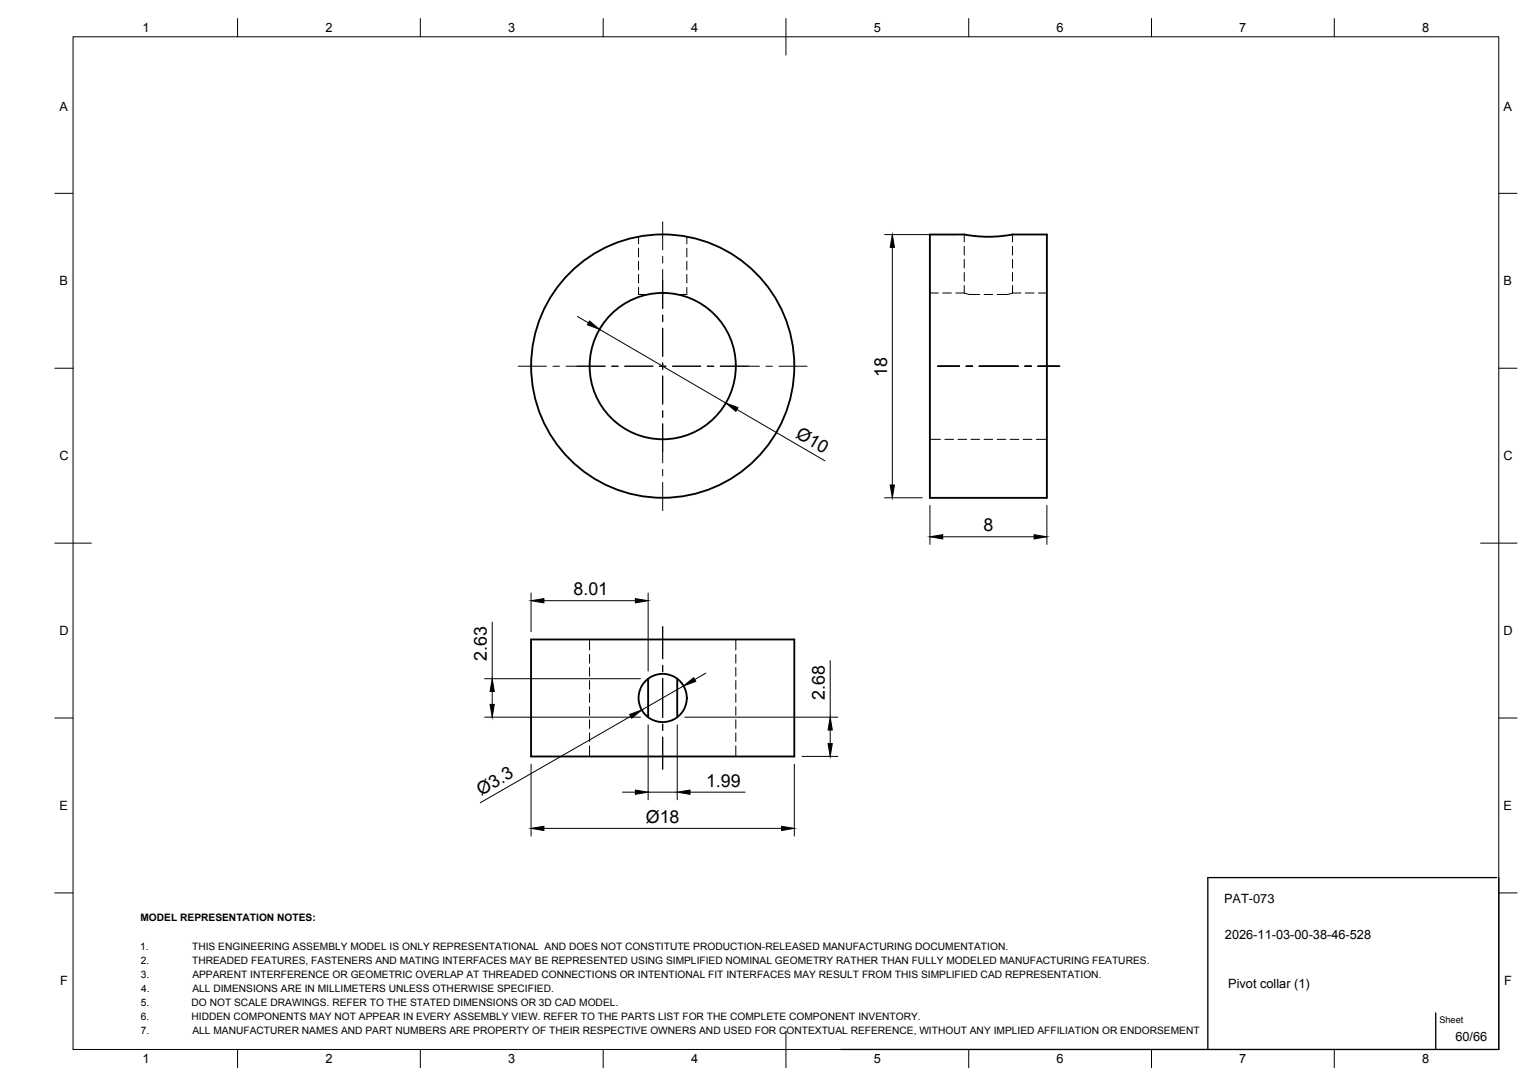
ISO-10303-21;
HEADER;
/* Generated by software containing ST-Developer
 * from STEP Tools, Inc. (www.steptools.com) 
 */

FILE_DESCRIPTION(
/* description */ ('Manual piston pump'),
/* implementation_level */ '2;1');

FILE_NAME(
/* name */ 'Pivot collar (1).step',
/* time_stamp */ '2026-11-02T16:54:23-08:00',
/* author */ (''),
/* organization */ (''),
/* preprocessor_version */ 'ST-DEVELOPER v20.2',
/* originating_system */ 'Autodesk Translation Framework v15.17.0.0',
/* authorisation */ '');

FILE_SCHEMA (('AUTOMOTIVE_DESIGN { 1 0 10303 214 3 1 1 }'));
ENDSEC;

DATA;
#10=MECHANICAL_DESIGN_GEOMETRIC_PRESENTATION_REPRESENTATION('',(#750),#19043);
#616=SHAPE_REPRESENTATION_RELATIONSHIP('SRR','None',#19366,#679);
#679=ADVANCED_BREP_SHAPE_REPRESENTATION('',(#818),#19033);
#750=STYLED_ITEM('',(#19661),#818);
#818=MANIFOLD_SOLID_BREP('Body1',#9538);
#1030=FACE_BOUND('',#2573,.T.);
#1031=FACE_BOUND('',#2575,.T.);
#1084=B_SPLINE_CURVE_WITH_KNOTS('',3,(#18479,#18480,#18481,#18482,#18483,
#18484),.UNSPECIFIED.,.F.,.F.,(4,2,4),(0.649292020015395,0.689320963667327,
0.7519713082482),.UNSPECIFIED.);
#1085=B_SPLINE_CURVE_WITH_KNOTS('',3,(#18488,#18489,#18490,#18491,#18492,
#18493),.UNSPECIFIED.,.F.,.F.,(4,2,4),(0.2506571027494,0.313307447330273,
0.353336390982205),.UNSPECIFIED.);
#1086=B_SPLINE_CURVE_WITH_KNOTS('',3,(#18494,#18495,#18496,#18497,#18498,
#18499),.UNSPECIFIED.,.F.,.F.,(4,2,4),(0.147977814516595,0.188006758168527,
0.2506571027494),.UNSPECIFIED.);
#1087=B_SPLINE_CURVE_WITH_KNOTS('',3,(#18500,#18501,#18502,#18503,#18504,
#18505),.UNSPECIFIED.,.F.,.F.,(4,2,4),(0.7519713082482,0.814621652829074,
0.854650596481005),.UNSPECIFIED.);
#1088=B_SPLINE_CURVE_WITH_KNOTS('',3,(#18509,#18510,#18511,#18512,#18513,
#18514,#18515,#18516,#18517,#18518),.UNSPECIFIED.,.F.,.F.,(4,2,2,2,4),(0.,
0.0623062782223143,0.124612556444629,0.186916384615149,0.249220212785669),
 .UNSPECIFIED.);
#1089=B_SPLINE_CURVE_WITH_KNOTS('',3,(#18520,#18521,#18522,#18523,#18524,
#18525,#18526,#18527,#18528,#18529),.UNSPECIFIED.,.F.,.F.,(4,2,2,2,4),(0.747660638357008,
0.809964466527528,0.872268294698049,0.934574572920363,0.996880851142677),
 .UNSPECIFIED.);
#1090=B_SPLINE_CURVE_WITH_KNOTS('',3,(#18530,#18531,#18532,#18533,#18534,
#18535,#18536,#18537,#18538,#18539,#18540,#18541,#18542,#18543,#18544,#18545,
#18546,#18547),.UNSPECIFIED.,.F.,.F.,(4,2,2,2,2,2,2,2,4),(0.249220212785669,
0.31152404095619,0.37382786912671,0.436134147349024,0.498440425571339,0.560746703793653,
0.623052982015967,0.685356810186488,0.747660638357008),.UNSPECIFIED.);
#1268=CYLINDRICAL_SURFACE('',#11326,0.165);
#1269=CYLINDRICAL_SURFACE('',#11329,0.5);
#1270=CYLINDRICAL_SURFACE('',#11332,0.9);
#1789=FACE_OUTER_BOUND('',#2567,.T.);
#1790=FACE_OUTER_BOUND('',#2568,.T.);
#1791=FACE_OUTER_BOUND('',#2569,.T.);
#1792=FACE_OUTER_BOUND('',#2570,.T.);
#1793=FACE_OUTER_BOUND('',#2571,.T.);
#1794=FACE_OUTER_BOUND('',#2572,.T.);
#1795=FACE_OUTER_BOUND('',#2574,.T.);
#2567=EDGE_LOOP('',(#8261,#8262));
#2568=EDGE_LOOP('',(#8263,#8264,#8265,#8266,#8267,#8268,#8269,#8270,#8271,
#8272,#8273));
#2569=EDGE_LOOP('',(#8274,#8275));
#2570=EDGE_LOOP('',(#8276,#8277,#8278,#8279,#8280,#8281,#8282,#8283,#8284,
#8285,#8286,#8287));
#2571=EDGE_LOOP('',(#8288,#8289,#8290,#8291,#8292,#8293,#8294,#8295,#8296));
#2572=EDGE_LOOP('',(#8297));
#2573=EDGE_LOOP('',(#8298));
#2574=EDGE_LOOP('',(#8299));
#2575=EDGE_LOOP('',(#8300));
#3094=CIRCLE('',#11325,0.165);
#3095=CIRCLE('',#11327,0.165);
#3096=CIRCLE('',#11330,0.5);
#3097=CIRCLE('',#11331,0.5);
#3098=CIRCLE('',#11333,0.9);
#3099=CIRCLE('',#11334,0.9);
#3655=LINE('',#18474,#4259);
#3656=LINE('',#18507,#4260);
#3657=LINE('',#18549,#4261);
#3658=LINE('',#18553,#4262);
#3659=LINE('',#18555,#4263);
#3660=LINE('',#18560,#4264);
#3661=LINE('',#18562,#4265);
#4259=VECTOR('',#14167,1.);
#4260=VECTOR('',#14174,0.165);
#4261=VECTOR('',#14177,1.);
#4262=VECTOR('',#14182,0.5);
#4263=VECTOR('',#14183,0.5);
#4264=VECTOR('',#14190,0.9);
#4265=VECTOR('',#14191,0.9);
#5021=VERTEX_POINT('',#18472);
#5022=VERTEX_POINT('',#18473);
#5023=VERTEX_POINT('',#18477);
#5024=VERTEX_POINT('',#18478);
#5025=VERTEX_POINT('',#18485);
#5026=VERTEX_POINT('',#18487);
#5027=VERTEX_POINT('',#18506);
#5028=VERTEX_POINT('',#18508);
#5029=VERTEX_POINT('',#18519);
#5030=VERTEX_POINT('',#18551);
#5031=VERTEX_POINT('',#18554);
#5032=VERTEX_POINT('',#18558);
#5033=VERTEX_POINT('',#18561);
#6117=EDGE_CURVE('',#5021,#5022,#3655,.T.);
#6118=EDGE_CURVE('',#5021,#5022,#3094,.T.);
#6119=EDGE_CURVE('',#5023,#5024,#1084,.T.);
#6120=EDGE_CURVE('',#5025,#5023,#3095,.T.);
#6121=EDGE_CURVE('',#5026,#5025,#1085,.T.);
#6122=EDGE_CURVE('',#5022,#5026,#1086,.T.);
#6123=EDGE_CURVE('',#5024,#5021,#1087,.T.);
#6124=EDGE_CURVE('',#5024,#5027,#3656,.T.);
#6125=EDGE_CURVE('',#5028,#5027,#1088,.T.);
#6126=EDGE_CURVE('',#5029,#5028,#1089,.T.);
#6127=EDGE_CURVE('',#5027,#5029,#1090,.T.);
#6128=EDGE_CURVE('',#5025,#5023,#3657,.T.);
#6129=EDGE_CURVE('',#5030,#5030,#3096,.T.);
#6130=EDGE_CURVE('',#5030,#5026,#3658,.T.);
#6131=EDGE_CURVE('',#5024,#5031,#3659,.T.);
#6132=EDGE_CURVE('',#5031,#5031,#3097,.T.);
#6133=EDGE_CURVE('',#5032,#5032,#3098,.T.);
#6134=EDGE_CURVE('',#5032,#5029,#3660,.T.);
#6135=EDGE_CURVE('',#5027,#5033,#3661,.T.);
#6136=EDGE_CURVE('',#5033,#5033,#3099,.T.);
#8261=ORIENTED_EDGE('',*,*,#6117,.F.);
#8262=ORIENTED_EDGE('',*,*,#6118,.T.);
#8263=ORIENTED_EDGE('',*,*,#6119,.F.);
#8264=ORIENTED_EDGE('',*,*,#6120,.F.);
#8265=ORIENTED_EDGE('',*,*,#6121,.F.);
#8266=ORIENTED_EDGE('',*,*,#6122,.F.);
#8267=ORIENTED_EDGE('',*,*,#6118,.F.);
#8268=ORIENTED_EDGE('',*,*,#6123,.F.);
#8269=ORIENTED_EDGE('',*,*,#6124,.T.);
#8270=ORIENTED_EDGE('',*,*,#6125,.F.);
#8271=ORIENTED_EDGE('',*,*,#6126,.F.);
#8272=ORIENTED_EDGE('',*,*,#6127,.F.);
#8273=ORIENTED_EDGE('',*,*,#6124,.F.);
#8274=ORIENTED_EDGE('',*,*,#6128,.F.);
#8275=ORIENTED_EDGE('',*,*,#6120,.T.);
#8276=ORIENTED_EDGE('',*,*,#6129,.F.);
#8277=ORIENTED_EDGE('',*,*,#6130,.T.);
#8278=ORIENTED_EDGE('',*,*,#6121,.T.);
#8279=ORIENTED_EDGE('',*,*,#6128,.T.);
#8280=ORIENTED_EDGE('',*,*,#6119,.T.);
#8281=ORIENTED_EDGE('',*,*,#6131,.T.);
#8282=ORIENTED_EDGE('',*,*,#6132,.T.);
#8283=ORIENTED_EDGE('',*,*,#6131,.F.);
#8284=ORIENTED_EDGE('',*,*,#6123,.T.);
#8285=ORIENTED_EDGE('',*,*,#6117,.T.);
#8286=ORIENTED_EDGE('',*,*,#6122,.T.);
#8287=ORIENTED_EDGE('',*,*,#6130,.F.);
#8288=ORIENTED_EDGE('',*,*,#6133,.F.);
#8289=ORIENTED_EDGE('',*,*,#6134,.T.);
#8290=ORIENTED_EDGE('',*,*,#6126,.T.);
#8291=ORIENTED_EDGE('',*,*,#6125,.T.);
#8292=ORIENTED_EDGE('',*,*,#6135,.T.);
#8293=ORIENTED_EDGE('',*,*,#6136,.T.);
#8294=ORIENTED_EDGE('',*,*,#6135,.F.);
#8295=ORIENTED_EDGE('',*,*,#6127,.T.);
#8296=ORIENTED_EDGE('',*,*,#6134,.F.);
#8297=ORIENTED_EDGE('',*,*,#6133,.T.);
#8298=ORIENTED_EDGE('',*,*,#6129,.T.);
#8299=ORIENTED_EDGE('',*,*,#6136,.F.);
#8300=ORIENTED_EDGE('',*,*,#6132,.F.);
#8848=PLANE('',#11324);
#8849=PLANE('',#11328);
#8850=PLANE('',#11335);
#8851=PLANE('',#11336);
#9394=ADVANCED_FACE('',(#1789),#8848,.T.);
#9395=ADVANCED_FACE('',(#1790),#1268,.F.);
#9396=ADVANCED_FACE('',(#1791),#8849,.T.);
#9397=ADVANCED_FACE('',(#1792),#1269,.F.);
#9398=ADVANCED_FACE('',(#1793),#1270,.T.);
#9399=ADVANCED_FACE('',(#1794,#1030),#8850,.T.);
#9400=ADVANCED_FACE('',(#1795,#1031),#8851,.F.);
#9538=CLOSED_SHELL('',(#9394,#9395,#9396,#9397,#9398,#9399,#9400));
#11323=AXIS2_PLACEMENT_3D('',#18470,#14163,#14164);
#11324=AXIS2_PLACEMENT_3D('',#18471,#14165,#14166);
#11325=AXIS2_PLACEMENT_3D('',#18475,#14168,#14169);
#11326=AXIS2_PLACEMENT_3D('',#18476,#14170,#14171);
#11327=AXIS2_PLACEMENT_3D('',#18486,#14172,#14173);
#11328=AXIS2_PLACEMENT_3D('',#18548,#14175,#14176);
#11329=AXIS2_PLACEMENT_3D('',#18550,#14178,#14179);
#11330=AXIS2_PLACEMENT_3D('',#18552,#14180,#14181);
#11331=AXIS2_PLACEMENT_3D('',#18556,#14184,#14185);
#11332=AXIS2_PLACEMENT_3D('',#18557,#14186,#14187);
#11333=AXIS2_PLACEMENT_3D('',#18559,#14188,#14189);
#11334=AXIS2_PLACEMENT_3D('',#18563,#14192,#14193);
#11335=AXIS2_PLACEMENT_3D('',#18564,#14194,#14195);
#11336=AXIS2_PLACEMENT_3D('',#18565,#14196,#14197);
#14163=DIRECTION('axis',(0.,0.,1.));
#14164=DIRECTION('refdir',(1.,0.,0.));
#14165=DIRECTION('center_axis',(0.,0.,1.));
#14166=DIRECTION('ref_axis',(1.,0.,0.));
#14167=DIRECTION('',(1.,0.,0.));
#14168=DIRECTION('center_axis',(0.,0.,1.));
#14169=DIRECTION('ref_axis',(1.,0.,0.));
#14170=DIRECTION('center_axis',(0.,0.,1.));
#14171=DIRECTION('ref_axis',(1.,0.,0.));
#14172=DIRECTION('center_axis',(0.,0.,1.));
#14173=DIRECTION('ref_axis',(1.,0.,0.));
#14174=DIRECTION('',(0.,0.,1.));
#14175=DIRECTION('center_axis',(0.,0.,1.));
#14176=DIRECTION('ref_axis',(1.,0.,0.));
#14177=DIRECTION('',(-1.,0.,0.));
#14178=DIRECTION('center_axis',(1.,0.,0.));
#14179=DIRECTION('ref_axis',(0.,0.,-1.));
#14180=DIRECTION('center_axis',(-1.,0.,0.));
#14181=DIRECTION('ref_axis',(0.,0.,-1.));
#14182=DIRECTION('',(-1.,0.,0.));
#14183=DIRECTION('',(-1.,0.,0.));
#14184=DIRECTION('center_axis',(-1.,0.,0.));
#14185=DIRECTION('ref_axis',(0.,0.,-1.));
#14186=DIRECTION('center_axis',(1.,0.,0.));
#14187=DIRECTION('ref_axis',(0.,0.,-1.));
#14188=DIRECTION('center_axis',(1.,0.,0.));
#14189=DIRECTION('ref_axis',(0.,0.,-1.));
#14190=DIRECTION('',(-1.,0.,0.));
#14191=DIRECTION('',(-1.,0.,0.));
#14192=DIRECTION('center_axis',(1.,0.,0.));
#14193=DIRECTION('ref_axis',(0.,0.,-1.));
#14194=DIRECTION('center_axis',(1.,0.,0.));
#14195=DIRECTION('ref_axis',(0.,0.,-1.));
#14196=DIRECTION('center_axis',(1.,0.,0.));
#14197=DIRECTION('ref_axis',(0.,0.,-1.));
#18470=CARTESIAN_POINT('',(0.,0.,0.));
#18471=CARTESIAN_POINT('Origin',(4.6,-4.,10.49));
#18472=CARTESIAN_POINT('',(4.46837553418911,-4.09949874371065,10.49));
#18473=CARTESIAN_POINT('',(4.73162446581089,-4.09949874371065,10.49));
#18474=CARTESIAN_POINT('',(4.2,-4.09949874371065,10.49));
#18475=CARTESIAN_POINT('Origin',(4.6,-4.,10.49));
#18476=CARTESIAN_POINT('Origin',(4.6,-4.,10.49));
#18477=CARTESIAN_POINT('',(4.46837553418911,-3.90050125628935,10.49));
#18478=CARTESIAN_POINT('',(4.435,-4.,10.5));
#18479=CARTESIAN_POINT('Ctrl Pts',(4.46837553418911,-3.90050125628935,10.49));
#18480=CARTESIAN_POINT('Ctrl Pts',(4.46012370297415,-3.91141740291719,10.4922166181135));
#18481=CARTESIAN_POINT('Ctrl Pts',(4.45304490097489,-3.92366776278637,10.4943120869024));
#18482=CARTESIAN_POINT('Ctrl Pts',(4.43920540953364,-3.95694557235505,10.4985632587304));
#18483=CARTESIAN_POINT('Ctrl Pts',(4.435,-3.97911655180638,10.5));
#18484=CARTESIAN_POINT('Ctrl Pts',(4.435,-4.,10.5));
#18485=CARTESIAN_POINT('',(4.73162446581089,-3.90050125628935,10.49));
#18486=CARTESIAN_POINT('Origin',(4.6,-4.,10.49));
#18487=CARTESIAN_POINT('',(4.765,-4.,10.5));
#18488=CARTESIAN_POINT('Ctrl Pts',(4.765,-4.,10.5));
#18489=CARTESIAN_POINT('Ctrl Pts',(4.765,-3.97911655180638,10.5));
#18490=CARTESIAN_POINT('Ctrl Pts',(4.76079459046636,-3.95694557235505,10.4985632587304));
#18491=CARTESIAN_POINT('Ctrl Pts',(4.74695509902511,-3.92366776278637,10.4943120869024));
#18492=CARTESIAN_POINT('Ctrl Pts',(4.73987629702585,-3.91141740291719,10.4922166181135));
#18493=CARTESIAN_POINT('Ctrl Pts',(4.73162446581089,-3.90050125628935,10.49));
#18494=CARTESIAN_POINT('Ctrl Pts',(4.73162446581089,-4.09949874371065,10.49));
#18495=CARTESIAN_POINT('Ctrl Pts',(4.73987629702585,-4.08858259708281,10.4922166181135));
#18496=CARTESIAN_POINT('Ctrl Pts',(4.74695509902511,-4.07633223721363,10.4943120869024));
#18497=CARTESIAN_POINT('Ctrl Pts',(4.76079459046636,-4.04305442764495,10.4985632587304));
#18498=CARTESIAN_POINT('Ctrl Pts',(4.765,-4.02088344819362,10.5));
#18499=CARTESIAN_POINT('Ctrl Pts',(4.765,-4.,10.5));
#18500=CARTESIAN_POINT('Ctrl Pts',(4.435,-4.,10.5));
#18501=CARTESIAN_POINT('Ctrl Pts',(4.435,-4.02088344819362,10.5));
#18502=CARTESIAN_POINT('Ctrl Pts',(4.43920540953364,-4.04305442764495,10.4985632587304));
#18503=CARTESIAN_POINT('Ctrl Pts',(4.45304490097489,-4.07633223721363,10.4943120869024));
#18504=CARTESIAN_POINT('Ctrl Pts',(4.46012370297415,-4.08858259708281,10.4922166181135));
#18505=CARTESIAN_POINT('Ctrl Pts',(4.46837553418911,-4.09949874371065,10.49));
#18506=CARTESIAN_POINT('',(4.435,-4.,10.9));
#18507=CARTESIAN_POINT('',(4.435,-4.,10.49));
#18508=CARTESIAN_POINT('',(4.6,-4.165,10.8847457261835));
#18509=CARTESIAN_POINT('Ctrl Pts',(4.6,-4.165,10.8847457261835));
#18510=CARTESIAN_POINT('Ctrl Pts',(4.57923124059256,-4.165,10.8847457261835));
#18511=CARTESIAN_POINT('Ctrl Pts',(4.55711110492665,-4.16083971900758,10.8855527595053));
#18512=CARTESIAN_POINT('Ctrl Pts',(4.51647293736623,-4.14398647021669,10.88844864815));
#18513=CARTESIAN_POINT('Ctrl Pts',(4.49795075602263,-4.13129599381419,10.8904936048516));
#18514=CARTESIAN_POINT('Ctrl Pts',(4.46870458121656,-4.10204981900812,10.8943172343239));
#18515=CARTESIAN_POINT('Ctrl Pts',(4.45601365401642,-4.08352739209068,10.8963470888995));
#18516=CARTESIAN_POINT('Ctrl Pts',(4.43916007816136,-4.04288837609341,10.8992082718606));
#18517=CARTESIAN_POINT('Ctrl Pts',(4.435,-4.02076794272351,10.9));
#18518=CARTESIAN_POINT('Ctrl Pts',(4.435,-4.,10.9));
#18519=CARTESIAN_POINT('',(4.765,-4.,10.9));
#18520=CARTESIAN_POINT('Ctrl Pts',(4.765,-4.,10.9));
#18521=CARTESIAN_POINT('Ctrl Pts',(4.765,-4.02076794272351,10.9));
#18522=CARTESIAN_POINT('Ctrl Pts',(4.76083992183864,-4.04288837609341,10.8992082718606));
#18523=CARTESIAN_POINT('Ctrl Pts',(4.74398634598358,-4.08352739209068,10.8963470888995));
#18524=CARTESIAN_POINT('Ctrl Pts',(4.73129541878344,-4.10204981900812,10.8943172343239));
#18525=CARTESIAN_POINT('Ctrl Pts',(4.70204924397737,-4.13129599381419,10.8904936048516));
#18526=CARTESIAN_POINT('Ctrl Pts',(4.68352706263377,-4.14398647021669,10.88844864815));
#18527=CARTESIAN_POINT('Ctrl Pts',(4.64288889507334,-4.16083971900758,10.8855527595053));
#18528=CARTESIAN_POINT('Ctrl Pts',(4.62076875940744,-4.165,10.8847457261835));
#18529=CARTESIAN_POINT('Ctrl Pts',(4.6,-4.165,10.8847457261835));
#18530=CARTESIAN_POINT('Ctrl Pts',(4.435,-4.,10.9));
#18531=CARTESIAN_POINT('Ctrl Pts',(4.435,-3.97923205727649,10.9));
#18532=CARTESIAN_POINT('Ctrl Pts',(4.43916007816136,-3.95711162390659,10.8992082718606));
#18533=CARTESIAN_POINT('Ctrl Pts',(4.45601365401642,-3.91647260790932,10.8963470888995));
#18534=CARTESIAN_POINT('Ctrl Pts',(4.46870458121656,-3.89795018099187,10.8943172343239));
#18535=CARTESIAN_POINT('Ctrl Pts',(4.49795075602263,-3.86870400618581,10.8904936048516));
#18536=CARTESIAN_POINT('Ctrl Pts',(4.51647293736623,-3.85601352978331,10.88844864815));
#18537=CARTESIAN_POINT('Ctrl Pts',(4.55711110492666,-3.83916028099242,10.8855527595053));
#18538=CARTESIAN_POINT('Ctrl Pts',(4.57923124059256,-3.835,10.8847457261835));
#18539=CARTESIAN_POINT('Ctrl Pts',(4.62076875940744,-3.835,10.8847457261835));
#18540=CARTESIAN_POINT('Ctrl Pts',(4.64288889507334,-3.83916028099242,10.8855527595053));
#18541=CARTESIAN_POINT('Ctrl Pts',(4.68352706263377,-3.85601352978331,10.88844864815));
#18542=CARTESIAN_POINT('Ctrl Pts',(4.70204924397737,-3.86870400618581,10.8904936048516));
#18543=CARTESIAN_POINT('Ctrl Pts',(4.73129541878344,-3.89795018099187,10.8943172343239));
#18544=CARTESIAN_POINT('Ctrl Pts',(4.74398634598358,-3.91647260790932,10.8963470888995));
#18545=CARTESIAN_POINT('Ctrl Pts',(4.76083992183864,-3.95711162390659,10.8992082718606));
#18546=CARTESIAN_POINT('Ctrl Pts',(4.765,-3.97923205727649,10.9));
#18547=CARTESIAN_POINT('Ctrl Pts',(4.765,-4.,10.9));
#18548=CARTESIAN_POINT('Origin',(4.6,-4.,10.49));
#18549=CARTESIAN_POINT('',(4.2,-3.90050125628935,10.49));
#18550=CARTESIAN_POINT('Origin',(4.2,-4.,10.));
#18551=CARTESIAN_POINT('',(5.,-4.,10.5));
#18552=CARTESIAN_POINT('Origin',(5.,-4.,10.));
#18553=CARTESIAN_POINT('',(4.2,-4.,10.5));
#18554=CARTESIAN_POINT('',(4.2,-4.,10.5));
#18555=CARTESIAN_POINT('',(4.2,-4.,10.5));
#18556=CARTESIAN_POINT('Origin',(4.2,-4.,10.));
#18557=CARTESIAN_POINT('Origin',(4.2,-4.,10.));
#18558=CARTESIAN_POINT('',(5.,-4.,10.9));
#18559=CARTESIAN_POINT('Origin',(5.,-4.,10.));
#18560=CARTESIAN_POINT('',(4.2,-4.,10.9));
#18561=CARTESIAN_POINT('',(4.2,-4.,10.9));
#18562=CARTESIAN_POINT('',(4.2,-4.,10.9));
#18563=CARTESIAN_POINT('Origin',(4.2,-4.,10.));
#18564=CARTESIAN_POINT('Origin',(5.,-4.,10.));
#18565=CARTESIAN_POINT('Origin',(4.2,-4.,10.));
#18962=UNCERTAINTY_MEASURE_WITH_UNIT(LENGTH_MEASURE(0.001),#19044,
'DISTANCE_ACCURACY_VALUE',
'Maximum model space distance between geometric entities at asserted c
onnectivities');
#18972=UNCERTAINTY_MEASURE_WITH_UNIT(LENGTH_MEASURE(0.001),#19044,
'DISTANCE_ACCURACY_VALUE',
'Maximum model space distance between geometric entities at asserted c
onnectivities');
#19033=(
GEOMETRIC_REPRESENTATION_CONTEXT(3)
GLOBAL_UNCERTAINTY_ASSIGNED_CONTEXT((#18962))
GLOBAL_UNIT_ASSIGNED_CONTEXT((#19044,#19046,#19047))
REPRESENTATION_CONTEXT('','3D')
);
#19043=(
GEOMETRIC_REPRESENTATION_CONTEXT(3)
GLOBAL_UNCERTAINTY_ASSIGNED_CONTEXT((#18972))
GLOBAL_UNIT_ASSIGNED_CONTEXT((#19044,#19046,#19047))
REPRESENTATION_CONTEXT('','3D')
);
#19044=(
LENGTH_UNIT()
NAMED_UNIT(*)
SI_UNIT(.CENTI.,.METRE.)
);
#19046=(
NAMED_UNIT(*)
PLANE_ANGLE_UNIT()
SI_UNIT($,.RADIAN.)
);
#19047=(
NAMED_UNIT(*)
SI_UNIT($,.STERADIAN.)
SOLID_ANGLE_UNIT()
);
#19108=SHAPE_DEFINITION_REPRESENTATION(#19265,#19366);
#19265=PRODUCT_DEFINITION_SHAPE('',$,#19437);
#19366=SHAPE_REPRESENTATION('',(#11323),#19033);
#19376=PRODUCT_DEFINITION_CONTEXT('part definition',#19588,'design');
#19437=PRODUCT_DEFINITION('2026-11-03-00-38-46-528','Pivot collar (1)',
#19507,#19376);
#19507=PRODUCT_DEFINITION_FORMATION('',$,#19650);
#19588=APPLICATION_CONTEXT(
'Core Data for Automotive Mechanical Design Process');
#19589=PRODUCT_CONTEXT('part definition',#19588,'mechanical');
#19650=PRODUCT('2026-11-03-00-38-46-528','Pivot collar (1)',
'Pivot collar',(#19589));
#19661=PRESENTATION_STYLE_ASSIGNMENT((#19667));
#19667=SURFACE_STYLE_USAGE(.BOTH.,#19673);
#19673=SURFACE_SIDE_STYLE('',(#19679));
#19679=SURFACE_STYLE_FILL_AREA(#19685);
#19685=FILL_AREA_STYLE('CAD Library Painted - Engineering blue',(#19691));
#19691=FILL_AREA_STYLE_COLOUR('CAD Library Painted - Engineering blue',
#19697);
#19697=COLOUR_RGB('CAD Library Painted - Engineering blue',0.12156862745098,
0.356862745098039,0.6);
ENDSEC;
END-ISO-10303-21;
